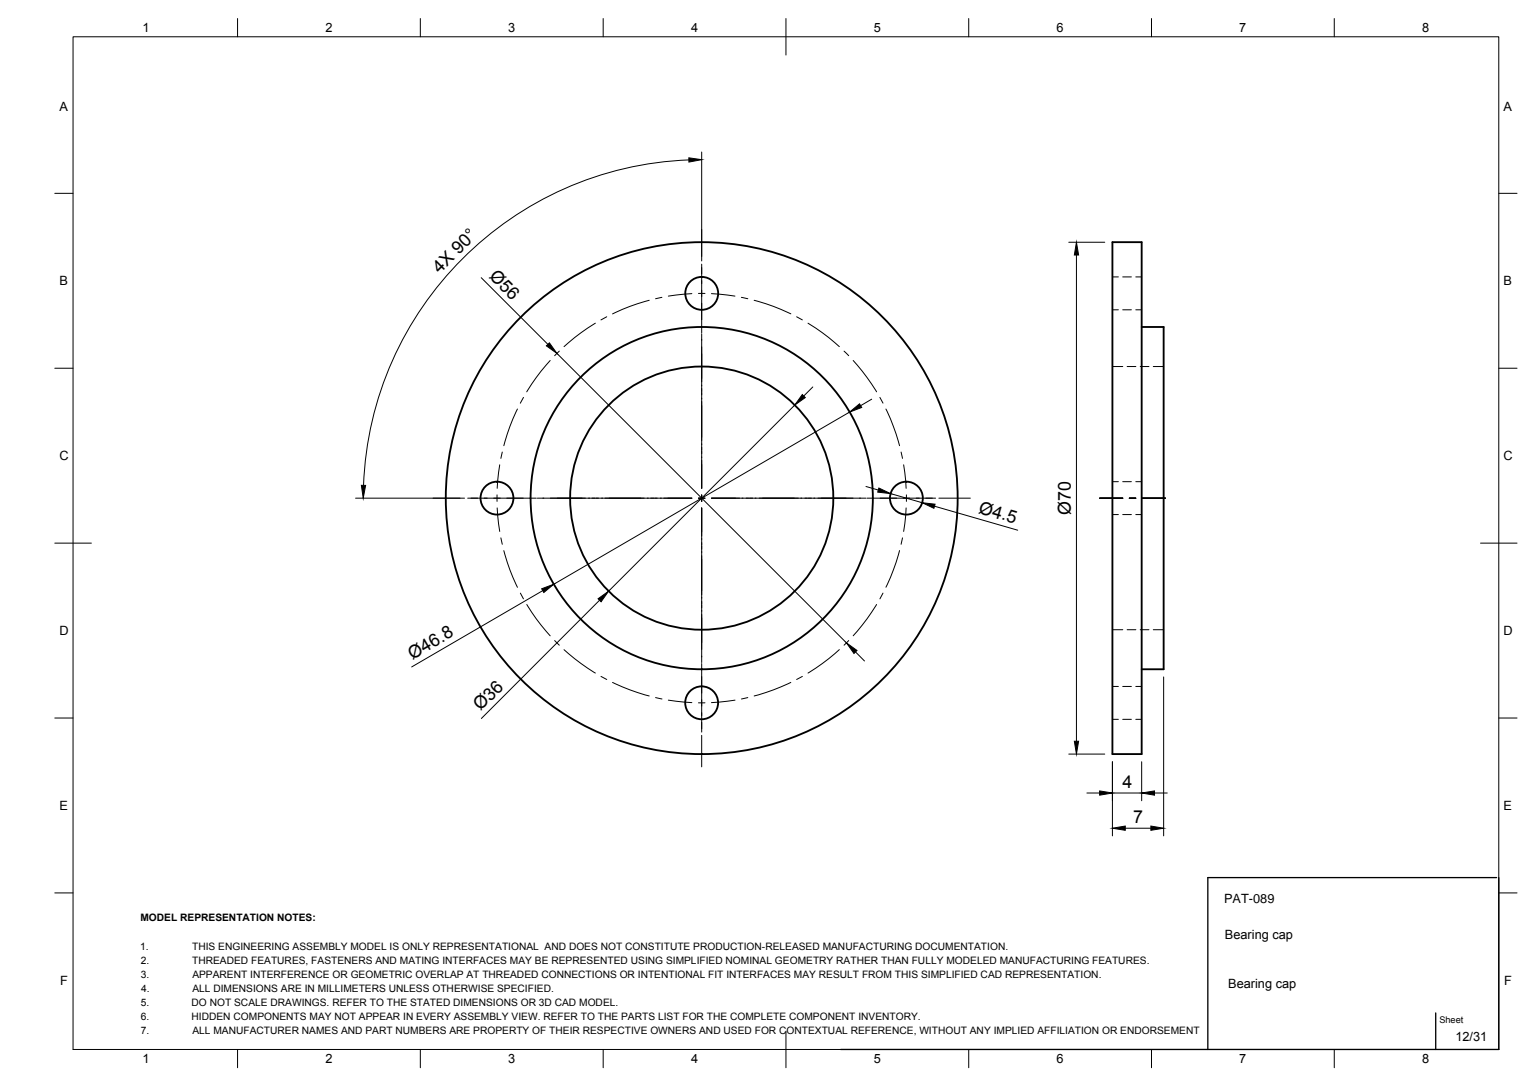
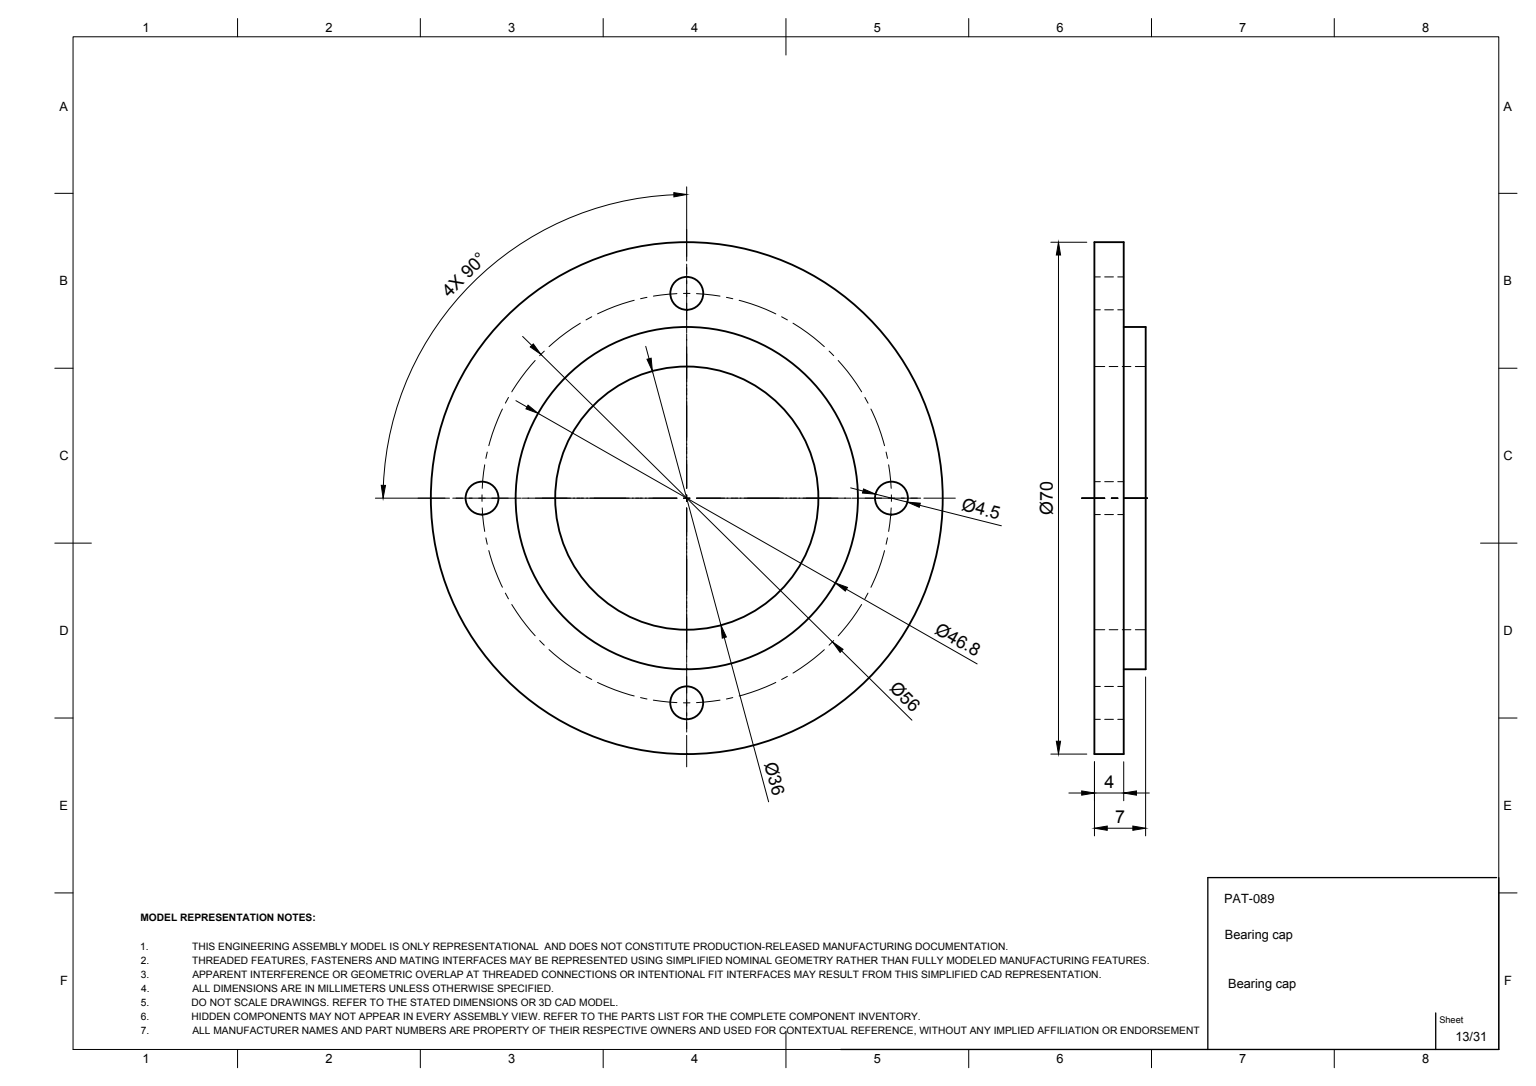
ISO-10303-21;
HEADER;
/* Generated by software containing ST-Developer
 * from STEP Tools, Inc. (www.steptools.com) 
 */

FILE_DESCRIPTION(
/* description */ ('Rotary union on bearing shaft'),
/* implementation_level */ '2;1');

FILE_NAME(
/* name */ 'Bearing cap.step',
/* time_stamp */ '2026-10-28T03:24:01-07:00',
/* author */ (''),
/* organization */ (''),
/* preprocessor_version */ 'ST-DEVELOPER v20.2',
/* originating_system */ 'Autodesk Translation Framework v15.17.0.0',
/* authorisation */ '');

FILE_SCHEMA (('AUTOMOTIVE_DESIGN { 1 0 10303 214 3 1 1 }'));
ENDSEC;

DATA;
#10=MECHANICAL_DESIGN_GEOMETRIC_PRESENTATION_REPRESENTATION('',(#320),#9448);
#266=SHAPE_REPRESENTATION_RELATIONSHIP('SRR','None',#9566,#293);
#293=ADVANCED_BREP_SHAPE_REPRESENTATION('',(#355),#9426);
#320=STYLED_ITEM('',(#9778),#355);
#355=MANIFOLD_SOLID_BREP('Body1',#4875);
#422=FACE_BOUND('',#1082,.T.);
#423=FACE_BOUND('',#1086,.T.);
#424=FACE_BOUND('',#1087,.T.);
#425=FACE_BOUND('',#1088,.T.);
#426=FACE_BOUND('',#1089,.T.);
#427=FACE_BOUND('',#1090,.T.);
#428=FACE_BOUND('',#1092,.T.);
#429=FACE_BOUND('',#1093,.T.);
#430=FACE_BOUND('',#1094,.T.);
#431=FACE_BOUND('',#1095,.T.);
#432=FACE_BOUND('',#1096,.T.);
#532=PLANE('',#5379);
#533=PLANE('',#5386);
#534=PLANE('',#5387);
#735=FACE_OUTER_BOUND('',#1076,.T.);
#736=FACE_OUTER_BOUND('',#1077,.T.);
#737=FACE_OUTER_BOUND('',#1078,.T.);
#738=FACE_OUTER_BOUND('',#1079,.T.);
#739=FACE_OUTER_BOUND('',#1080,.T.);
#740=FACE_OUTER_BOUND('',#1081,.T.);
#741=FACE_OUTER_BOUND('',#1083,.T.);
#742=FACE_OUTER_BOUND('',#1084,.T.);
#743=FACE_OUTER_BOUND('',#1085,.T.);
#744=FACE_OUTER_BOUND('',#1091,.T.);
#1076=EDGE_LOOP('',(#3591,#3592,#3593,#3594));
#1077=EDGE_LOOP('',(#3595,#3596,#3597,#3598));
#1078=EDGE_LOOP('',(#3599,#3600,#3601,#3602));
#1079=EDGE_LOOP('',(#3603,#3604,#3605,#3606));
#1080=EDGE_LOOP('',(#3607,#3608,#3609,#3610));
#1081=EDGE_LOOP('',(#3611));
#1082=EDGE_LOOP('',(#3612));
#1083=EDGE_LOOP('',(#3613,#3614,#3615,#3616));
#1084=EDGE_LOOP('',(#3617,#3618,#3619,#3620));
#1085=EDGE_LOOP('',(#3621));
#1086=EDGE_LOOP('',(#3622));
#1087=EDGE_LOOP('',(#3623));
#1088=EDGE_LOOP('',(#3624));
#1089=EDGE_LOOP('',(#3625));
#1090=EDGE_LOOP('',(#3626));
#1091=EDGE_LOOP('',(#3627));
#1092=EDGE_LOOP('',(#3628));
#1093=EDGE_LOOP('',(#3629));
#1094=EDGE_LOOP('',(#3630));
#1095=EDGE_LOOP('',(#3631));
#1096=EDGE_LOOP('',(#3632));
#1444=LINE('',#7887,#1764);
#1445=LINE('',#7893,#1765);
#1446=LINE('',#7899,#1766);
#1447=LINE('',#7905,#1767);
#1448=LINE('',#7911,#1768);
#1449=LINE('',#7918,#1769);
#1450=LINE('',#7924,#1770);
#1764=VECTOR('',#6235,0.225);
#1765=VECTOR('',#6242,0.225);
#1766=VECTOR('',#6249,0.225);
#1767=VECTOR('',#6256,0.225);
#1768=VECTOR('',#6263,2.34);
#1769=VECTOR('',#6272,1.8);
#1770=VECTOR('',#6279,3.5);
#2072=CIRCLE('',#5365,0.225);
#2073=CIRCLE('',#5366,0.225);
#2074=CIRCLE('',#5368,0.225);
#2075=CIRCLE('',#5369,0.225);
#2076=CIRCLE('',#5371,0.225);
#2077=CIRCLE('',#5372,0.225);
#2078=CIRCLE('',#5374,0.225);
#2079=CIRCLE('',#5375,0.225);
#2080=CIRCLE('',#5377,2.34);
#2081=CIRCLE('',#5378,2.34);
#2082=CIRCLE('',#5380,1.8);
#2083=CIRCLE('',#5382,1.8);
#2084=CIRCLE('',#5384,3.5);
#2085=CIRCLE('',#5385,3.5);
#2360=VERTEX_POINT('',#7884);
#2361=VERTEX_POINT('',#7886);
#2362=VERTEX_POINT('',#7890);
#2363=VERTEX_POINT('',#7892);
#2364=VERTEX_POINT('',#7896);
#2365=VERTEX_POINT('',#7898);
#2366=VERTEX_POINT('',#7902);
#2367=VERTEX_POINT('',#7904);
#2368=VERTEX_POINT('',#7908);
#2369=VERTEX_POINT('',#7910);
#2370=VERTEX_POINT('',#7914);
#2371=VERTEX_POINT('',#7917);
#2372=VERTEX_POINT('',#7921);
#2373=VERTEX_POINT('',#7923);
#2823=EDGE_CURVE('',#2360,#2360,#2072,.T.);
#2824=EDGE_CURVE('',#2360,#2361,#1444,.T.);
#2825=EDGE_CURVE('',#2361,#2361,#2073,.T.);
#2826=EDGE_CURVE('',#2362,#2362,#2074,.T.);
#2827=EDGE_CURVE('',#2362,#2363,#1445,.T.);
#2828=EDGE_CURVE('',#2363,#2363,#2075,.T.);
#2829=EDGE_CURVE('',#2364,#2364,#2076,.T.);
#2830=EDGE_CURVE('',#2364,#2365,#1446,.T.);
#2831=EDGE_CURVE('',#2365,#2365,#2077,.T.);
#2832=EDGE_CURVE('',#2366,#2366,#2078,.T.);
#2833=EDGE_CURVE('',#2366,#2367,#1447,.T.);
#2834=EDGE_CURVE('',#2367,#2367,#2079,.T.);
#2835=EDGE_CURVE('',#2368,#2368,#2080,.T.);
#2836=EDGE_CURVE('',#2368,#2369,#1448,.T.);
#2837=EDGE_CURVE('',#2369,#2369,#2081,.T.);
#2838=EDGE_CURVE('',#2370,#2370,#2082,.T.);
#2839=EDGE_CURVE('',#2370,#2371,#1449,.T.);
#2840=EDGE_CURVE('',#2371,#2371,#2083,.T.);
#2841=EDGE_CURVE('',#2372,#2372,#2084,.T.);
#2842=EDGE_CURVE('',#2372,#2373,#1450,.T.);
#2843=EDGE_CURVE('',#2373,#2373,#2085,.T.);
#3591=ORIENTED_EDGE('',*,*,#2823,.F.);
#3592=ORIENTED_EDGE('',*,*,#2824,.T.);
#3593=ORIENTED_EDGE('',*,*,#2825,.F.);
#3594=ORIENTED_EDGE('',*,*,#2824,.F.);
#3595=ORIENTED_EDGE('',*,*,#2826,.F.);
#3596=ORIENTED_EDGE('',*,*,#2827,.T.);
#3597=ORIENTED_EDGE('',*,*,#2828,.F.);
#3598=ORIENTED_EDGE('',*,*,#2827,.F.);
#3599=ORIENTED_EDGE('',*,*,#2829,.F.);
#3600=ORIENTED_EDGE('',*,*,#2830,.T.);
#3601=ORIENTED_EDGE('',*,*,#2831,.F.);
#3602=ORIENTED_EDGE('',*,*,#2830,.F.);
#3603=ORIENTED_EDGE('',*,*,#2832,.F.);
#3604=ORIENTED_EDGE('',*,*,#2833,.T.);
#3605=ORIENTED_EDGE('',*,*,#2834,.F.);
#3606=ORIENTED_EDGE('',*,*,#2833,.F.);
#3607=ORIENTED_EDGE('',*,*,#2835,.F.);
#3608=ORIENTED_EDGE('',*,*,#2836,.T.);
#3609=ORIENTED_EDGE('',*,*,#2837,.F.);
#3610=ORIENTED_EDGE('',*,*,#2836,.F.);
#3611=ORIENTED_EDGE('',*,*,#2835,.T.);
#3612=ORIENTED_EDGE('',*,*,#2838,.T.);
#3613=ORIENTED_EDGE('',*,*,#2838,.F.);
#3614=ORIENTED_EDGE('',*,*,#2839,.T.);
#3615=ORIENTED_EDGE('',*,*,#2840,.T.);
#3616=ORIENTED_EDGE('',*,*,#2839,.F.);
#3617=ORIENTED_EDGE('',*,*,#2841,.F.);
#3618=ORIENTED_EDGE('',*,*,#2842,.T.);
#3619=ORIENTED_EDGE('',*,*,#2843,.T.);
#3620=ORIENTED_EDGE('',*,*,#2842,.F.);
#3621=ORIENTED_EDGE('',*,*,#2841,.T.);
#3622=ORIENTED_EDGE('',*,*,#2837,.T.);
#3623=ORIENTED_EDGE('',*,*,#2834,.T.);
#3624=ORIENTED_EDGE('',*,*,#2831,.T.);
#3625=ORIENTED_EDGE('',*,*,#2828,.T.);
#3626=ORIENTED_EDGE('',*,*,#2825,.T.);
#3627=ORIENTED_EDGE('',*,*,#2843,.F.);
#3628=ORIENTED_EDGE('',*,*,#2840,.F.);
#3629=ORIENTED_EDGE('',*,*,#2832,.T.);
#3630=ORIENTED_EDGE('',*,*,#2829,.T.);
#3631=ORIENTED_EDGE('',*,*,#2826,.T.);
#3632=ORIENTED_EDGE('',*,*,#2823,.T.);
#4511=CYLINDRICAL_SURFACE('',#5364,0.225);
#4512=CYLINDRICAL_SURFACE('',#5367,0.225);
#4513=CYLINDRICAL_SURFACE('',#5370,0.225);
#4514=CYLINDRICAL_SURFACE('',#5373,0.225);
#4515=CYLINDRICAL_SURFACE('',#5376,2.34);
#4516=CYLINDRICAL_SURFACE('',#5381,1.8);
#4517=CYLINDRICAL_SURFACE('',#5383,3.5);
#4648=ADVANCED_FACE('',(#735),#4511,.F.);
#4649=ADVANCED_FACE('',(#736),#4512,.F.);
#4650=ADVANCED_FACE('',(#737),#4513,.F.);
#4651=ADVANCED_FACE('',(#738),#4514,.F.);
#4652=ADVANCED_FACE('',(#739),#4515,.T.);
#4653=ADVANCED_FACE('',(#740,#422),#532,.T.);
#4654=ADVANCED_FACE('',(#741),#4516,.F.);
#4655=ADVANCED_FACE('',(#742),#4517,.T.);
#4656=ADVANCED_FACE('',(#743,#423,#424,#425,#426,#427),#533,.T.);
#4657=ADVANCED_FACE('',(#744,#428,#429,#430,#431,#432),#534,.F.);
#4875=CLOSED_SHELL('',(#4648,#4649,#4650,#4651,#4652,#4653,#4654,#4655,
#4656,#4657));
#5363=AXIS2_PLACEMENT_3D('',#7882,#6229,#6230);
#5364=AXIS2_PLACEMENT_3D('',#7883,#6231,#6232);
#5365=AXIS2_PLACEMENT_3D('',#7885,#6233,#6234);
#5366=AXIS2_PLACEMENT_3D('',#7888,#6236,#6237);
#5367=AXIS2_PLACEMENT_3D('',#7889,#6238,#6239);
#5368=AXIS2_PLACEMENT_3D('',#7891,#6240,#6241);
#5369=AXIS2_PLACEMENT_3D('',#7894,#6243,#6244);
#5370=AXIS2_PLACEMENT_3D('',#7895,#6245,#6246);
#5371=AXIS2_PLACEMENT_3D('',#7897,#6247,#6248);
#5372=AXIS2_PLACEMENT_3D('',#7900,#6250,#6251);
#5373=AXIS2_PLACEMENT_3D('',#7901,#6252,#6253);
#5374=AXIS2_PLACEMENT_3D('',#7903,#6254,#6255);
#5375=AXIS2_PLACEMENT_3D('',#7906,#6257,#6258);
#5376=AXIS2_PLACEMENT_3D('',#7907,#6259,#6260);
#5377=AXIS2_PLACEMENT_3D('',#7909,#6261,#6262);
#5378=AXIS2_PLACEMENT_3D('',#7912,#6264,#6265);
#5379=AXIS2_PLACEMENT_3D('',#7913,#6266,#6267);
#5380=AXIS2_PLACEMENT_3D('',#7915,#6268,#6269);
#5381=AXIS2_PLACEMENT_3D('',#7916,#6270,#6271);
#5382=AXIS2_PLACEMENT_3D('',#7919,#6273,#6274);
#5383=AXIS2_PLACEMENT_3D('',#7920,#6275,#6276);
#5384=AXIS2_PLACEMENT_3D('',#7922,#6277,#6278);
#5385=AXIS2_PLACEMENT_3D('',#7925,#6280,#6281);
#5386=AXIS2_PLACEMENT_3D('',#7926,#6282,#6283);
#5387=AXIS2_PLACEMENT_3D('',#7927,#6284,#6285);
#6229=DIRECTION('axis',(0.,0.,1.));
#6230=DIRECTION('refdir',(1.,0.,0.));
#6231=DIRECTION('center_axis',(0.,1.,0.));
#6232=DIRECTION('ref_axis',(1.,0.,0.));
#6233=DIRECTION('center_axis',(0.,1.,0.));
#6234=DIRECTION('ref_axis',(1.,0.,0.));
#6235=DIRECTION('',(0.,1.,0.));
#6236=DIRECTION('center_axis',(0.,-1.,0.));
#6237=DIRECTION('ref_axis',(1.,0.,0.));
#6238=DIRECTION('center_axis',(0.,1.,0.));
#6239=DIRECTION('ref_axis',(1.,0.,0.));
#6240=DIRECTION('center_axis',(0.,1.,0.));
#6241=DIRECTION('ref_axis',(1.,0.,0.));
#6242=DIRECTION('',(0.,1.,0.));
#6243=DIRECTION('center_axis',(0.,-1.,0.));
#6244=DIRECTION('ref_axis',(1.,0.,0.));
#6245=DIRECTION('center_axis',(0.,1.,0.));
#6246=DIRECTION('ref_axis',(1.,0.,0.));
#6247=DIRECTION('center_axis',(0.,1.,0.));
#6248=DIRECTION('ref_axis',(1.,0.,0.));
#6249=DIRECTION('',(0.,1.,0.));
#6250=DIRECTION('center_axis',(0.,-1.,0.));
#6251=DIRECTION('ref_axis',(1.,0.,0.));
#6252=DIRECTION('center_axis',(0.,1.,0.));
#6253=DIRECTION('ref_axis',(1.,0.,0.));
#6254=DIRECTION('center_axis',(0.,1.,0.));
#6255=DIRECTION('ref_axis',(1.,0.,0.));
#6256=DIRECTION('',(0.,1.,0.));
#6257=DIRECTION('center_axis',(0.,-1.,0.));
#6258=DIRECTION('ref_axis',(1.,0.,0.));
#6259=DIRECTION('center_axis',(0.,1.,0.));
#6260=DIRECTION('ref_axis',(1.,0.,0.));
#6261=DIRECTION('center_axis',(0.,1.,0.));
#6262=DIRECTION('ref_axis',(1.,0.,0.));
#6263=DIRECTION('',(0.,-1.,0.));
#6264=DIRECTION('center_axis',(0.,-1.,0.));
#6265=DIRECTION('ref_axis',(1.,0.,0.));
#6266=DIRECTION('center_axis',(0.,1.,0.));
#6267=DIRECTION('ref_axis',(1.,0.,0.));
#6268=DIRECTION('center_axis',(0.,-1.,0.));
#6269=DIRECTION('ref_axis',(1.,0.,0.));
#6270=DIRECTION('center_axis',(0.,1.,0.));
#6271=DIRECTION('ref_axis',(1.,0.,0.));
#6272=DIRECTION('',(0.,-1.,0.));
#6273=DIRECTION('center_axis',(0.,-1.,0.));
#6274=DIRECTION('ref_axis',(1.,0.,0.));
#6275=DIRECTION('center_axis',(0.,1.,0.));
#6276=DIRECTION('ref_axis',(1.,0.,0.));
#6277=DIRECTION('center_axis',(0.,1.,0.));
#6278=DIRECTION('ref_axis',(1.,0.,0.));
#6279=DIRECTION('',(0.,-1.,0.));
#6280=DIRECTION('center_axis',(0.,1.,0.));
#6281=DIRECTION('ref_axis',(1.,0.,0.));
#6282=DIRECTION('center_axis',(0.,1.,0.));
#6283=DIRECTION('ref_axis',(1.,0.,0.));
#6284=DIRECTION('center_axis',(0.,1.,0.));
#6285=DIRECTION('ref_axis',(1.,0.,0.));
#7882=CARTESIAN_POINT('',(0.,0.,0.));
#7883=CARTESIAN_POINT('Origin',(-2.8,-0.5,4.5));
#7884=CARTESIAN_POINT('',(-3.025,-0.4,4.5));
#7885=CARTESIAN_POINT('Origin',(-2.8,-0.4,4.5));
#7886=CARTESIAN_POINT('',(-3.025,0.,4.5));
#7887=CARTESIAN_POINT('',(-3.025,-0.5,4.5));
#7888=CARTESIAN_POINT('Origin',(-2.8,0.,4.5));
#7889=CARTESIAN_POINT('Origin',(1.71450551880629E-16,-0.5,7.3));
#7890=CARTESIAN_POINT('',(-0.225,-0.4,7.3));
#7891=CARTESIAN_POINT('Origin',(1.71450551880629E-16,-0.4,7.3));
#7892=CARTESIAN_POINT('',(-0.225,0.,7.3));
#7893=CARTESIAN_POINT('',(-0.225,-0.5,7.3));
#7894=CARTESIAN_POINT('Origin',(1.71450551880629E-16,0.,7.3));
#7895=CARTESIAN_POINT('Origin',(2.8,-0.5,4.5));
#7896=CARTESIAN_POINT('',(2.575,-0.4,4.5));
#7897=CARTESIAN_POINT('Origin',(2.8,-0.4,4.5));
#7898=CARTESIAN_POINT('',(2.575,0.,4.5));
#7899=CARTESIAN_POINT('',(2.575,-0.5,4.5));
#7900=CARTESIAN_POINT('Origin',(2.8,0.,4.5));
#7901=CARTESIAN_POINT('Origin',(-5.14351655641888E-16,-0.5,1.7));
#7902=CARTESIAN_POINT('',(-0.225000000000001,-0.4,1.7));
#7903=CARTESIAN_POINT('Origin',(-5.14351655641888E-16,-0.4,1.7));
#7904=CARTESIAN_POINT('',(-0.225000000000001,0.,1.7));
#7905=CARTESIAN_POINT('',(-0.225000000000001,-0.5,1.7));
#7906=CARTESIAN_POINT('Origin',(-5.14351655641888E-16,0.,1.7));
#7907=CARTESIAN_POINT('Origin',(0.,0.,4.5));
#7908=CARTESIAN_POINT('',(-2.34,0.3,4.5));
#7909=CARTESIAN_POINT('Origin',(0.,0.3,4.5));
#7910=CARTESIAN_POINT('',(-2.34,0.,4.5));
#7911=CARTESIAN_POINT('',(-2.34,0.,4.5));
#7912=CARTESIAN_POINT('Origin',(0.,0.,4.5));
#7913=CARTESIAN_POINT('Origin',(0.,0.3,4.5));
#7914=CARTESIAN_POINT('',(-1.8,0.3,4.5));
#7915=CARTESIAN_POINT('Origin',(0.,0.3,4.5));
#7916=CARTESIAN_POINT('Origin',(0.,-0.4,4.5));
#7917=CARTESIAN_POINT('',(-1.8,-0.4,4.5));
#7918=CARTESIAN_POINT('',(-1.8,-0.4,4.5));
#7919=CARTESIAN_POINT('Origin',(0.,-0.4,4.5));
#7920=CARTESIAN_POINT('Origin',(0.,-0.4,4.5));
#7921=CARTESIAN_POINT('',(-3.5,0.,4.5));
#7922=CARTESIAN_POINT('Origin',(0.,0.,4.5));
#7923=CARTESIAN_POINT('',(-3.5,-0.4,4.5));
#7924=CARTESIAN_POINT('',(-3.5,-0.4,4.5));
#7925=CARTESIAN_POINT('Origin',(0.,-0.4,4.5));
#7926=CARTESIAN_POINT('Origin',(0.,0.,4.5));
#7927=CARTESIAN_POINT('Origin',(0.,-0.4,4.5));
#9394=UNCERTAINTY_MEASURE_WITH_UNIT(LENGTH_MEASURE(0.001),#9449,
'DISTANCE_ACCURACY_VALUE',
'Maximum model space distance between geometric entities at asserted c
onnectivities');
#9416=UNCERTAINTY_MEASURE_WITH_UNIT(LENGTH_MEASURE(0.001),#9449,
'DISTANCE_ACCURACY_VALUE',
'Maximum model space distance between geometric entities at asserted c
onnectivities');
#9426=(
GEOMETRIC_REPRESENTATION_CONTEXT(3)
GLOBAL_UNCERTAINTY_ASSIGNED_CONTEXT((#9394))
GLOBAL_UNIT_ASSIGNED_CONTEXT((#9449,#9451,#9452))
REPRESENTATION_CONTEXT('','3D')
);
#9448=(
GEOMETRIC_REPRESENTATION_CONTEXT(3)
GLOBAL_UNCERTAINTY_ASSIGNED_CONTEXT((#9416))
GLOBAL_UNIT_ASSIGNED_CONTEXT((#9449,#9451,#9452))
REPRESENTATION_CONTEXT('','3D')
);
#9449=(
LENGTH_UNIT()
NAMED_UNIT(*)
SI_UNIT(.CENTI.,.METRE.)
);
#9451=(
NAMED_UNIT(*)
PLANE_ANGLE_UNIT()
SI_UNIT($,.RADIAN.)
);
#9452=(
NAMED_UNIT(*)
SI_UNIT($,.STERADIAN.)
SOLID_ANGLE_UNIT()
);
#9462=SHAPE_DEFINITION_REPRESENTATION(#9493,#9566);
#9493=PRODUCT_DEFINITION_SHAPE('',$,#9598);
#9566=SHAPE_REPRESENTATION('',(#5363),#9426);
#9588=PRODUCT_DEFINITION_CONTEXT('part definition',#9683,'design');
#9598=PRODUCT_DEFINITION('Bearing cap','Bearing cap',#9629,#9588);
#9629=PRODUCT_DEFINITION_FORMATION('',$,#9694);
#9683=APPLICATION_CONTEXT(
'Core Data for Automotive Mechanical Design Process');
#9684=PRODUCT_CONTEXT('part definition',#9683,'mechanical');
#9694=PRODUCT('Bearing cap','Bearing cap','Bearing cap',(#9684));
#9772=COLOUR_RGB('Grey',0.48,0.52,0.57);
#9773=FILL_AREA_STYLE_COLOUR('',#9772);
#9774=FILL_AREA_STYLE('',(#9773));
#9775=SURFACE_STYLE_FILL_AREA(#9774);
#9776=SURFACE_SIDE_STYLE('',(#9775));
#9777=SURFACE_STYLE_USAGE(.BOTH.,#9776);
#9778=PRESENTATION_STYLE_ASSIGNMENT((#9777));
ENDSEC;
END-ISO-10303-21;
